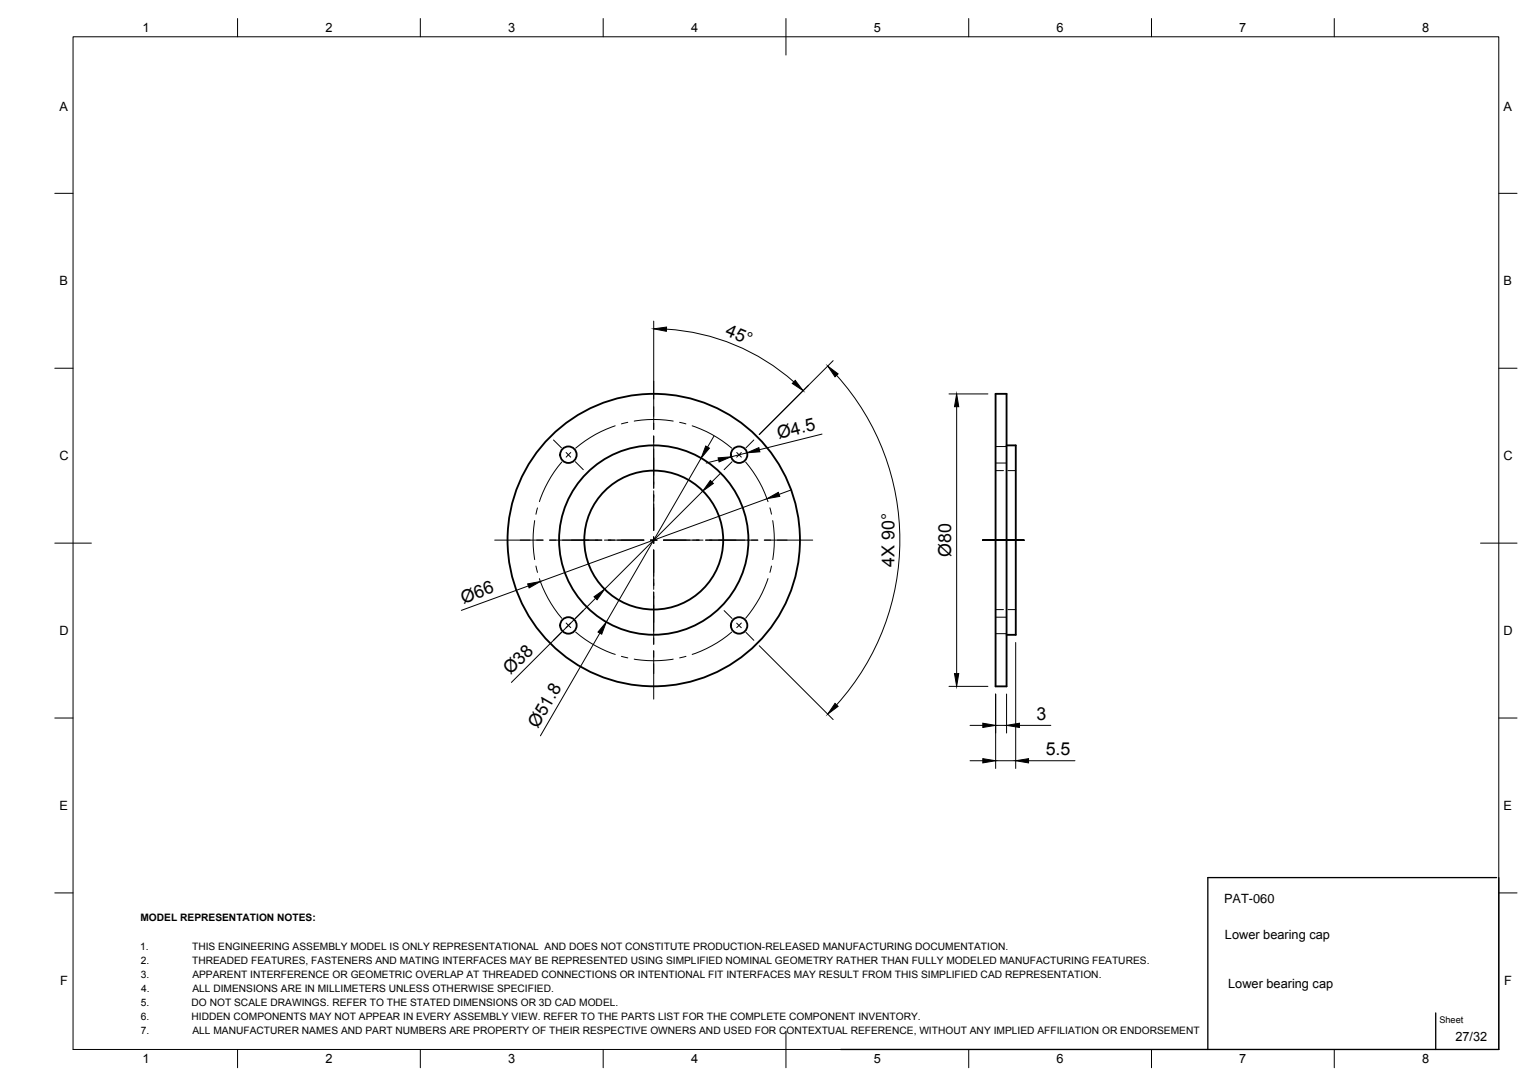
ISO-10303-21;
HEADER;
/* Generated by software containing ST-Developer
 * from STEP Tools, Inc. (www.steptools.com) 
 */

FILE_DESCRIPTION(
/* description */ ('Indexing fixture plate with plunger'),
/* implementation_level */ '2;1');

FILE_NAME(
/* name */ 'Lower bearing cap.step',
/* time_stamp */ '2026-10-28T03:23:41-07:00',
/* author */ (''),
/* organization */ (''),
/* preprocessor_version */ 'ST-DEVELOPER v20.2',
/* originating_system */ 'Autodesk Translation Framework v15.17.0.0',
/* authorisation */ '');

FILE_SCHEMA (('AUTOMOTIVE_DESIGN { 1 0 10303 214 3 1 1 }'));
ENDSEC;

DATA;
#10=MECHANICAL_DESIGN_GEOMETRIC_PRESENTATION_REPRESENTATION('',(#347),#10020);
#284=SHAPE_REPRESENTATION_RELATIONSHIP('SRR','None',#10160,#311);
#311=ADVANCED_BREP_SHAPE_REPRESENTATION('',(#382),#10013);
#347=STYLED_ITEM('',(#10368),#382);
#382=MANIFOLD_SOLID_BREP('Body1',#4602);
#484=FACE_BOUND('',#1272,.T.);
#485=FACE_BOUND('',#1276,.T.);
#486=FACE_BOUND('',#1277,.T.);
#487=FACE_BOUND('',#1278,.T.);
#488=FACE_BOUND('',#1279,.T.);
#489=FACE_BOUND('',#1280,.T.);
#490=FACE_BOUND('',#1282,.T.);
#491=FACE_BOUND('',#1283,.T.);
#492=FACE_BOUND('',#1284,.T.);
#493=FACE_BOUND('',#1285,.T.);
#494=FACE_BOUND('',#1286,.T.);
#637=PLANE('',#5394);
#638=PLANE('',#5401);
#639=PLANE('',#5402);
#883=FACE_OUTER_BOUND('',#1266,.T.);
#884=FACE_OUTER_BOUND('',#1267,.T.);
#885=FACE_OUTER_BOUND('',#1268,.T.);
#886=FACE_OUTER_BOUND('',#1269,.T.);
#887=FACE_OUTER_BOUND('',#1270,.T.);
#888=FACE_OUTER_BOUND('',#1271,.T.);
#889=FACE_OUTER_BOUND('',#1273,.T.);
#890=FACE_OUTER_BOUND('',#1274,.T.);
#891=FACE_OUTER_BOUND('',#1275,.T.);
#892=FACE_OUTER_BOUND('',#1281,.T.);
#1266=EDGE_LOOP('',(#3853,#3854,#3855,#3856));
#1267=EDGE_LOOP('',(#3857,#3858,#3859,#3860));
#1268=EDGE_LOOP('',(#3861,#3862,#3863,#3864));
#1269=EDGE_LOOP('',(#3865,#3866,#3867,#3868));
#1270=EDGE_LOOP('',(#3869,#3870,#3871,#3872));
#1271=EDGE_LOOP('',(#3873));
#1272=EDGE_LOOP('',(#3874));
#1273=EDGE_LOOP('',(#3875,#3876,#3877,#3878));
#1274=EDGE_LOOP('',(#3879,#3880,#3881,#3882));
#1275=EDGE_LOOP('',(#3883));
#1276=EDGE_LOOP('',(#3884));
#1277=EDGE_LOOP('',(#3885));
#1278=EDGE_LOOP('',(#3886));
#1279=EDGE_LOOP('',(#3887));
#1280=EDGE_LOOP('',(#3888));
#1281=EDGE_LOOP('',(#3889));
#1282=EDGE_LOOP('',(#3890));
#1283=EDGE_LOOP('',(#3891));
#1284=EDGE_LOOP('',(#3892));
#1285=EDGE_LOOP('',(#3893));
#1286=EDGE_LOOP('',(#3894));
#1534=LINE('',#9534,#1754);
#1535=LINE('',#9540,#1755);
#1536=LINE('',#9546,#1756);
#1537=LINE('',#9552,#1757);
#1538=LINE('',#9558,#1758);
#1539=LINE('',#9565,#1759);
#1540=LINE('',#9571,#1760);
#1754=VECTOR('',#6663,0.225);
#1755=VECTOR('',#6670,0.225);
#1756=VECTOR('',#6677,0.225);
#1757=VECTOR('',#6684,0.225);
#1758=VECTOR('',#6691,2.59);
#1759=VECTOR('',#6700,1.9);
#1760=VECTOR('',#6707,4.);
#2061=CIRCLE('',#5380,0.225);
#2062=CIRCLE('',#5381,0.225);
#2063=CIRCLE('',#5383,0.225);
#2064=CIRCLE('',#5384,0.225);
#2065=CIRCLE('',#5386,0.225);
#2066=CIRCLE('',#5387,0.225);
#2067=CIRCLE('',#5389,0.225);
#2068=CIRCLE('',#5390,0.225);
#2069=CIRCLE('',#5392,2.59);
#2070=CIRCLE('',#5393,2.59);
#2071=CIRCLE('',#5395,1.9);
#2072=CIRCLE('',#5397,1.9);
#2073=CIRCLE('',#5399,4.);
#2074=CIRCLE('',#5400,4.);
#2408=VERTEX_POINT('',#9531);
#2409=VERTEX_POINT('',#9533);
#2410=VERTEX_POINT('',#9537);
#2411=VERTEX_POINT('',#9539);
#2412=VERTEX_POINT('',#9543);
#2413=VERTEX_POINT('',#9545);
#2414=VERTEX_POINT('',#9549);
#2415=VERTEX_POINT('',#9551);
#2416=VERTEX_POINT('',#9555);
#2417=VERTEX_POINT('',#9557);
#2418=VERTEX_POINT('',#9561);
#2419=VERTEX_POINT('',#9564);
#2420=VERTEX_POINT('',#9568);
#2421=VERTEX_POINT('',#9570);
#2906=EDGE_CURVE('',#2408,#2408,#2061,.T.);
#2907=EDGE_CURVE('',#2408,#2409,#1534,.T.);
#2908=EDGE_CURVE('',#2409,#2409,#2062,.T.);
#2909=EDGE_CURVE('',#2410,#2410,#2063,.T.);
#2910=EDGE_CURVE('',#2410,#2411,#1535,.T.);
#2911=EDGE_CURVE('',#2411,#2411,#2064,.T.);
#2912=EDGE_CURVE('',#2412,#2412,#2065,.T.);
#2913=EDGE_CURVE('',#2412,#2413,#1536,.T.);
#2914=EDGE_CURVE('',#2413,#2413,#2066,.T.);
#2915=EDGE_CURVE('',#2414,#2414,#2067,.T.);
#2916=EDGE_CURVE('',#2414,#2415,#1537,.T.);
#2917=EDGE_CURVE('',#2415,#2415,#2068,.T.);
#2918=EDGE_CURVE('',#2416,#2416,#2069,.T.);
#2919=EDGE_CURVE('',#2416,#2417,#1538,.T.);
#2920=EDGE_CURVE('',#2417,#2417,#2070,.T.);
#2921=EDGE_CURVE('',#2418,#2418,#2071,.T.);
#2922=EDGE_CURVE('',#2418,#2419,#1539,.T.);
#2923=EDGE_CURVE('',#2419,#2419,#2072,.T.);
#2924=EDGE_CURVE('',#2420,#2420,#2073,.T.);
#2925=EDGE_CURVE('',#2420,#2421,#1540,.T.);
#2926=EDGE_CURVE('',#2421,#2421,#2074,.T.);
#3853=ORIENTED_EDGE('',*,*,#2906,.F.);
#3854=ORIENTED_EDGE('',*,*,#2907,.T.);
#3855=ORIENTED_EDGE('',*,*,#2908,.F.);
#3856=ORIENTED_EDGE('',*,*,#2907,.F.);
#3857=ORIENTED_EDGE('',*,*,#2909,.F.);
#3858=ORIENTED_EDGE('',*,*,#2910,.T.);
#3859=ORIENTED_EDGE('',*,*,#2911,.F.);
#3860=ORIENTED_EDGE('',*,*,#2910,.F.);
#3861=ORIENTED_EDGE('',*,*,#2912,.F.);
#3862=ORIENTED_EDGE('',*,*,#2913,.T.);
#3863=ORIENTED_EDGE('',*,*,#2914,.F.);
#3864=ORIENTED_EDGE('',*,*,#2913,.F.);
#3865=ORIENTED_EDGE('',*,*,#2915,.F.);
#3866=ORIENTED_EDGE('',*,*,#2916,.T.);
#3867=ORIENTED_EDGE('',*,*,#2917,.F.);
#3868=ORIENTED_EDGE('',*,*,#2916,.F.);
#3869=ORIENTED_EDGE('',*,*,#2918,.F.);
#3870=ORIENTED_EDGE('',*,*,#2919,.T.);
#3871=ORIENTED_EDGE('',*,*,#2920,.F.);
#3872=ORIENTED_EDGE('',*,*,#2919,.F.);
#3873=ORIENTED_EDGE('',*,*,#2918,.T.);
#3874=ORIENTED_EDGE('',*,*,#2921,.T.);
#3875=ORIENTED_EDGE('',*,*,#2921,.F.);
#3876=ORIENTED_EDGE('',*,*,#2922,.T.);
#3877=ORIENTED_EDGE('',*,*,#2923,.T.);
#3878=ORIENTED_EDGE('',*,*,#2922,.F.);
#3879=ORIENTED_EDGE('',*,*,#2924,.F.);
#3880=ORIENTED_EDGE('',*,*,#2925,.T.);
#3881=ORIENTED_EDGE('',*,*,#2926,.T.);
#3882=ORIENTED_EDGE('',*,*,#2925,.F.);
#3883=ORIENTED_EDGE('',*,*,#2924,.T.);
#3884=ORIENTED_EDGE('',*,*,#2920,.T.);
#3885=ORIENTED_EDGE('',*,*,#2917,.T.);
#3886=ORIENTED_EDGE('',*,*,#2914,.T.);
#3887=ORIENTED_EDGE('',*,*,#2911,.T.);
#3888=ORIENTED_EDGE('',*,*,#2908,.T.);
#3889=ORIENTED_EDGE('',*,*,#2926,.F.);
#3890=ORIENTED_EDGE('',*,*,#2923,.F.);
#3891=ORIENTED_EDGE('',*,*,#2915,.T.);
#3892=ORIENTED_EDGE('',*,*,#2912,.T.);
#3893=ORIENTED_EDGE('',*,*,#2909,.T.);
#3894=ORIENTED_EDGE('',*,*,#2906,.T.);
#4251=CYLINDRICAL_SURFACE('',#5379,0.225);
#4252=CYLINDRICAL_SURFACE('',#5382,0.225);
#4253=CYLINDRICAL_SURFACE('',#5385,0.225);
#4254=CYLINDRICAL_SURFACE('',#5388,0.225);
#4255=CYLINDRICAL_SURFACE('',#5391,2.59);
#4256=CYLINDRICAL_SURFACE('',#5396,1.9);
#4257=CYLINDRICAL_SURFACE('',#5398,4.);
#4498=ADVANCED_FACE('',(#883),#4251,.F.);
#4499=ADVANCED_FACE('',(#884),#4252,.F.);
#4500=ADVANCED_FACE('',(#885),#4253,.F.);
#4501=ADVANCED_FACE('',(#886),#4254,.F.);
#4502=ADVANCED_FACE('',(#887),#4255,.T.);
#4503=ADVANCED_FACE('',(#888,#484),#637,.T.);
#4504=ADVANCED_FACE('',(#889),#4256,.F.);
#4505=ADVANCED_FACE('',(#890),#4257,.T.);
#4506=ADVANCED_FACE('',(#891,#485,#486,#487,#488,#489),#638,.T.);
#4507=ADVANCED_FACE('',(#892,#490,#491,#492,#493,#494),#639,.F.);
#4602=CLOSED_SHELL('',(#4498,#4499,#4500,#4501,#4502,#4503,#4504,#4505,
#4506,#4507));
#5378=AXIS2_PLACEMENT_3D('',#9529,#6657,#6658);
#5379=AXIS2_PLACEMENT_3D('',#9530,#6659,#6660);
#5380=AXIS2_PLACEMENT_3D('',#9532,#6661,#6662);
#5381=AXIS2_PLACEMENT_3D('',#9535,#6664,#6665);
#5382=AXIS2_PLACEMENT_3D('',#9536,#6666,#6667);
#5383=AXIS2_PLACEMENT_3D('',#9538,#6668,#6669);
#5384=AXIS2_PLACEMENT_3D('',#9541,#6671,#6672);
#5385=AXIS2_PLACEMENT_3D('',#9542,#6673,#6674);
#5386=AXIS2_PLACEMENT_3D('',#9544,#6675,#6676);
#5387=AXIS2_PLACEMENT_3D('',#9547,#6678,#6679);
#5388=AXIS2_PLACEMENT_3D('',#9548,#6680,#6681);
#5389=AXIS2_PLACEMENT_3D('',#9550,#6682,#6683);
#5390=AXIS2_PLACEMENT_3D('',#9553,#6685,#6686);
#5391=AXIS2_PLACEMENT_3D('',#9554,#6687,#6688);
#5392=AXIS2_PLACEMENT_3D('',#9556,#6689,#6690);
#5393=AXIS2_PLACEMENT_3D('',#9559,#6692,#6693);
#5394=AXIS2_PLACEMENT_3D('',#9560,#6694,#6695);
#5395=AXIS2_PLACEMENT_3D('',#9562,#6696,#6697);
#5396=AXIS2_PLACEMENT_3D('',#9563,#6698,#6699);
#5397=AXIS2_PLACEMENT_3D('',#9566,#6701,#6702);
#5398=AXIS2_PLACEMENT_3D('',#9567,#6703,#6704);
#5399=AXIS2_PLACEMENT_3D('',#9569,#6705,#6706);
#5400=AXIS2_PLACEMENT_3D('',#9572,#6708,#6709);
#5401=AXIS2_PLACEMENT_3D('',#9573,#6710,#6711);
#5402=AXIS2_PLACEMENT_3D('',#9574,#6712,#6713);
#6657=DIRECTION('axis',(0.,0.,1.));
#6658=DIRECTION('refdir',(1.,0.,0.));
#6659=DIRECTION('center_axis',(0.,0.,1.));
#6660=DIRECTION('ref_axis',(1.,0.,0.));
#6661=DIRECTION('center_axis',(0.,0.,1.));
#6662=DIRECTION('ref_axis',(1.,0.,0.));
#6663=DIRECTION('',(0.,0.,1.));
#6664=DIRECTION('center_axis',(0.,0.,-1.));
#6665=DIRECTION('ref_axis',(1.,0.,0.));
#6666=DIRECTION('center_axis',(0.,0.,1.));
#6667=DIRECTION('ref_axis',(1.,0.,0.));
#6668=DIRECTION('center_axis',(0.,0.,1.));
#6669=DIRECTION('ref_axis',(1.,0.,0.));
#6670=DIRECTION('',(0.,0.,1.));
#6671=DIRECTION('center_axis',(0.,0.,-1.));
#6672=DIRECTION('ref_axis',(1.,0.,0.));
#6673=DIRECTION('center_axis',(0.,0.,1.));
#6674=DIRECTION('ref_axis',(1.,0.,0.));
#6675=DIRECTION('center_axis',(0.,0.,1.));
#6676=DIRECTION('ref_axis',(1.,0.,0.));
#6677=DIRECTION('',(0.,0.,1.));
#6678=DIRECTION('center_axis',(0.,0.,-1.));
#6679=DIRECTION('ref_axis',(1.,0.,0.));
#6680=DIRECTION('center_axis',(0.,0.,1.));
#6681=DIRECTION('ref_axis',(1.,0.,0.));
#6682=DIRECTION('center_axis',(0.,0.,1.));
#6683=DIRECTION('ref_axis',(1.,0.,0.));
#6684=DIRECTION('',(0.,0.,1.));
#6685=DIRECTION('center_axis',(0.,0.,-1.));
#6686=DIRECTION('ref_axis',(1.,0.,0.));
#6687=DIRECTION('center_axis',(0.,0.,1.));
#6688=DIRECTION('ref_axis',(1.,0.,0.));
#6689=DIRECTION('center_axis',(0.,0.,1.));
#6690=DIRECTION('ref_axis',(1.,0.,0.));
#6691=DIRECTION('',(0.,0.,-1.));
#6692=DIRECTION('center_axis',(0.,0.,-1.));
#6693=DIRECTION('ref_axis',(1.,0.,0.));
#6694=DIRECTION('center_axis',(0.,0.,1.));
#6695=DIRECTION('ref_axis',(1.,0.,0.));
#6696=DIRECTION('center_axis',(0.,0.,-1.));
#6697=DIRECTION('ref_axis',(1.,0.,0.));
#6698=DIRECTION('center_axis',(0.,0.,1.));
#6699=DIRECTION('ref_axis',(1.,0.,0.));
#6700=DIRECTION('',(0.,0.,-1.));
#6701=DIRECTION('center_axis',(0.,0.,-1.));
#6702=DIRECTION('ref_axis',(1.,0.,0.));
#6703=DIRECTION('center_axis',(0.,0.,1.));
#6704=DIRECTION('ref_axis',(1.,0.,0.));
#6705=DIRECTION('center_axis',(0.,0.,1.));
#6706=DIRECTION('ref_axis',(1.,0.,0.));
#6707=DIRECTION('',(0.,0.,-1.));
#6708=DIRECTION('center_axis',(0.,0.,1.));
#6709=DIRECTION('ref_axis',(1.,0.,0.));
#6710=DIRECTION('center_axis',(0.,0.,1.));
#6711=DIRECTION('ref_axis',(1.,0.,0.));
#6712=DIRECTION('center_axis',(0.,0.,1.));
#6713=DIRECTION('ref_axis',(1.,0.,0.));
#9529=CARTESIAN_POINT('',(0.,0.,0.));
#9530=CARTESIAN_POINT('Origin',(-2.33345237791561,-2.33345237791561,2.6));
#9531=CARTESIAN_POINT('',(-2.55845237791561,-2.33345237791561,2.7));
#9532=CARTESIAN_POINT('Origin',(-2.33345237791561,-2.33345237791561,2.7));
#9533=CARTESIAN_POINT('',(-2.55845237791561,-2.33345237791561,3.));
#9534=CARTESIAN_POINT('',(-2.55845237791561,-2.33345237791561,2.6));
#9535=CARTESIAN_POINT('Origin',(-2.33345237791561,-2.33345237791561,3.));
#9536=CARTESIAN_POINT('Origin',(-2.33345237791561,2.33345237791561,2.6));
#9537=CARTESIAN_POINT('',(-2.55845237791561,2.33345237791561,2.7));
#9538=CARTESIAN_POINT('Origin',(-2.33345237791561,2.33345237791561,2.7));
#9539=CARTESIAN_POINT('',(-2.55845237791561,2.33345237791561,3.));
#9540=CARTESIAN_POINT('',(-2.55845237791561,2.33345237791561,2.6));
#9541=CARTESIAN_POINT('Origin',(-2.33345237791561,2.33345237791561,3.));
#9542=CARTESIAN_POINT('Origin',(2.33345237791561,2.33345237791561,2.6));
#9543=CARTESIAN_POINT('',(2.10845237791561,2.33345237791561,2.7));
#9544=CARTESIAN_POINT('Origin',(2.33345237791561,2.33345237791561,2.7));
#9545=CARTESIAN_POINT('',(2.10845237791561,2.33345237791561,3.));
#9546=CARTESIAN_POINT('',(2.10845237791561,2.33345237791561,2.6));
#9547=CARTESIAN_POINT('Origin',(2.33345237791561,2.33345237791561,3.));
#9548=CARTESIAN_POINT('Origin',(2.33345237791561,-2.33345237791561,2.6));
#9549=CARTESIAN_POINT('',(2.10845237791561,-2.33345237791561,2.7));
#9550=CARTESIAN_POINT('Origin',(2.33345237791561,-2.33345237791561,2.7));
#9551=CARTESIAN_POINT('',(2.10845237791561,-2.33345237791561,3.));
#9552=CARTESIAN_POINT('',(2.10845237791561,-2.33345237791561,2.6));
#9553=CARTESIAN_POINT('Origin',(2.33345237791561,-2.33345237791561,3.));
#9554=CARTESIAN_POINT('Origin',(0.,0.,3.));
#9555=CARTESIAN_POINT('',(-2.59,-3.17183520979164E-16,3.25));
#9556=CARTESIAN_POINT('Origin',(0.,0.,3.25));
#9557=CARTESIAN_POINT('',(-2.59,-3.17183520979164E-16,3.));
#9558=CARTESIAN_POINT('',(-2.59,-3.17183520979164E-16,3.));
#9559=CARTESIAN_POINT('Origin',(0.,0.,3.));
#9560=CARTESIAN_POINT('Origin',(0.,0.,3.25));
#9561=CARTESIAN_POINT('',(-1.9,-2.32682891837997E-16,3.25));
#9562=CARTESIAN_POINT('Origin',(0.,0.,3.25));
#9563=CARTESIAN_POINT('Origin',(0.,0.,2.7));
#9564=CARTESIAN_POINT('',(-1.9,-2.32682891837997E-16,2.7));
#9565=CARTESIAN_POINT('',(-1.9,-2.32682891837997E-16,2.7));
#9566=CARTESIAN_POINT('Origin',(0.,0.,2.7));
#9567=CARTESIAN_POINT('Origin',(0.,0.,2.7));
#9568=CARTESIAN_POINT('',(-4.,-4.89858719658941E-16,3.));
#9569=CARTESIAN_POINT('Origin',(0.,0.,3.));
#9570=CARTESIAN_POINT('',(-4.,-4.89858719658941E-16,2.7));
#9571=CARTESIAN_POINT('',(-4.,-4.89858719658941E-16,2.7));
#9572=CARTESIAN_POINT('Origin',(0.,0.,2.7));
#9573=CARTESIAN_POINT('Origin',(0.,0.,3.));
#9574=CARTESIAN_POINT('Origin',(0.,0.,2.7));
#9980=UNCERTAINTY_MEASURE_WITH_UNIT(LENGTH_MEASURE(0.001),#10021,
'DISTANCE_ACCURACY_VALUE',
'Maximum model space distance between geometric entities at asserted c
onnectivities');
#9987=UNCERTAINTY_MEASURE_WITH_UNIT(LENGTH_MEASURE(0.001),#10021,
'DISTANCE_ACCURACY_VALUE',
'Maximum model space distance between geometric entities at asserted c
onnectivities');
#10013=(
GEOMETRIC_REPRESENTATION_CONTEXT(3)
GLOBAL_UNCERTAINTY_ASSIGNED_CONTEXT((#9980))
GLOBAL_UNIT_ASSIGNED_CONTEXT((#10021,#10023,#10024))
REPRESENTATION_CONTEXT('','3D')
);
#10020=(
GEOMETRIC_REPRESENTATION_CONTEXT(3)
GLOBAL_UNCERTAINTY_ASSIGNED_CONTEXT((#9987))
GLOBAL_UNIT_ASSIGNED_CONTEXT((#10021,#10023,#10024))
REPRESENTATION_CONTEXT('','3D')
);
#10021=(
LENGTH_UNIT()
NAMED_UNIT(*)
SI_UNIT(.CENTI.,.METRE.)
);
#10023=(
NAMED_UNIT(*)
PLANE_ANGLE_UNIT()
SI_UNIT($,.RADIAN.)
);
#10024=(
NAMED_UNIT(*)
SI_UNIT($,.STERADIAN.)
SOLID_ANGLE_UNIT()
);
#10050=SHAPE_DEFINITION_REPRESENTATION(#10087,#10160);
#10087=PRODUCT_DEFINITION_SHAPE('',$,#10193);
#10160=SHAPE_REPRESENTATION('',(#5378),#10013);
#10167=PRODUCT_DEFINITION_CONTEXT('part definition',#10265,'design');
#10193=PRODUCT_DEFINITION('Lower bearing cap','Lower bearing cap',#10225,
#10167);
#10225=PRODUCT_DEFINITION_FORMATION('',$,#10292);
#10265=APPLICATION_CONTEXT(
'Core Data for Automotive Mechanical Design Process');
#10266=PRODUCT_CONTEXT('part definition',#10265,'mechanical');
#10292=PRODUCT('Lower bearing cap','Lower bearing cap',
'Lower bearing cap',(#10266));
#10362=COLOUR_RGB('Grey',0.48,0.52,0.57);
#10363=FILL_AREA_STYLE_COLOUR('',#10362);
#10364=FILL_AREA_STYLE('',(#10363));
#10365=SURFACE_STYLE_FILL_AREA(#10364);
#10366=SURFACE_SIDE_STYLE('',(#10365));
#10367=SURFACE_STYLE_USAGE(.BOTH.,#10366);
#10368=PRESENTATION_STYLE_ASSIGNMENT((#10367));
ENDSEC;
END-ISO-10303-21;
